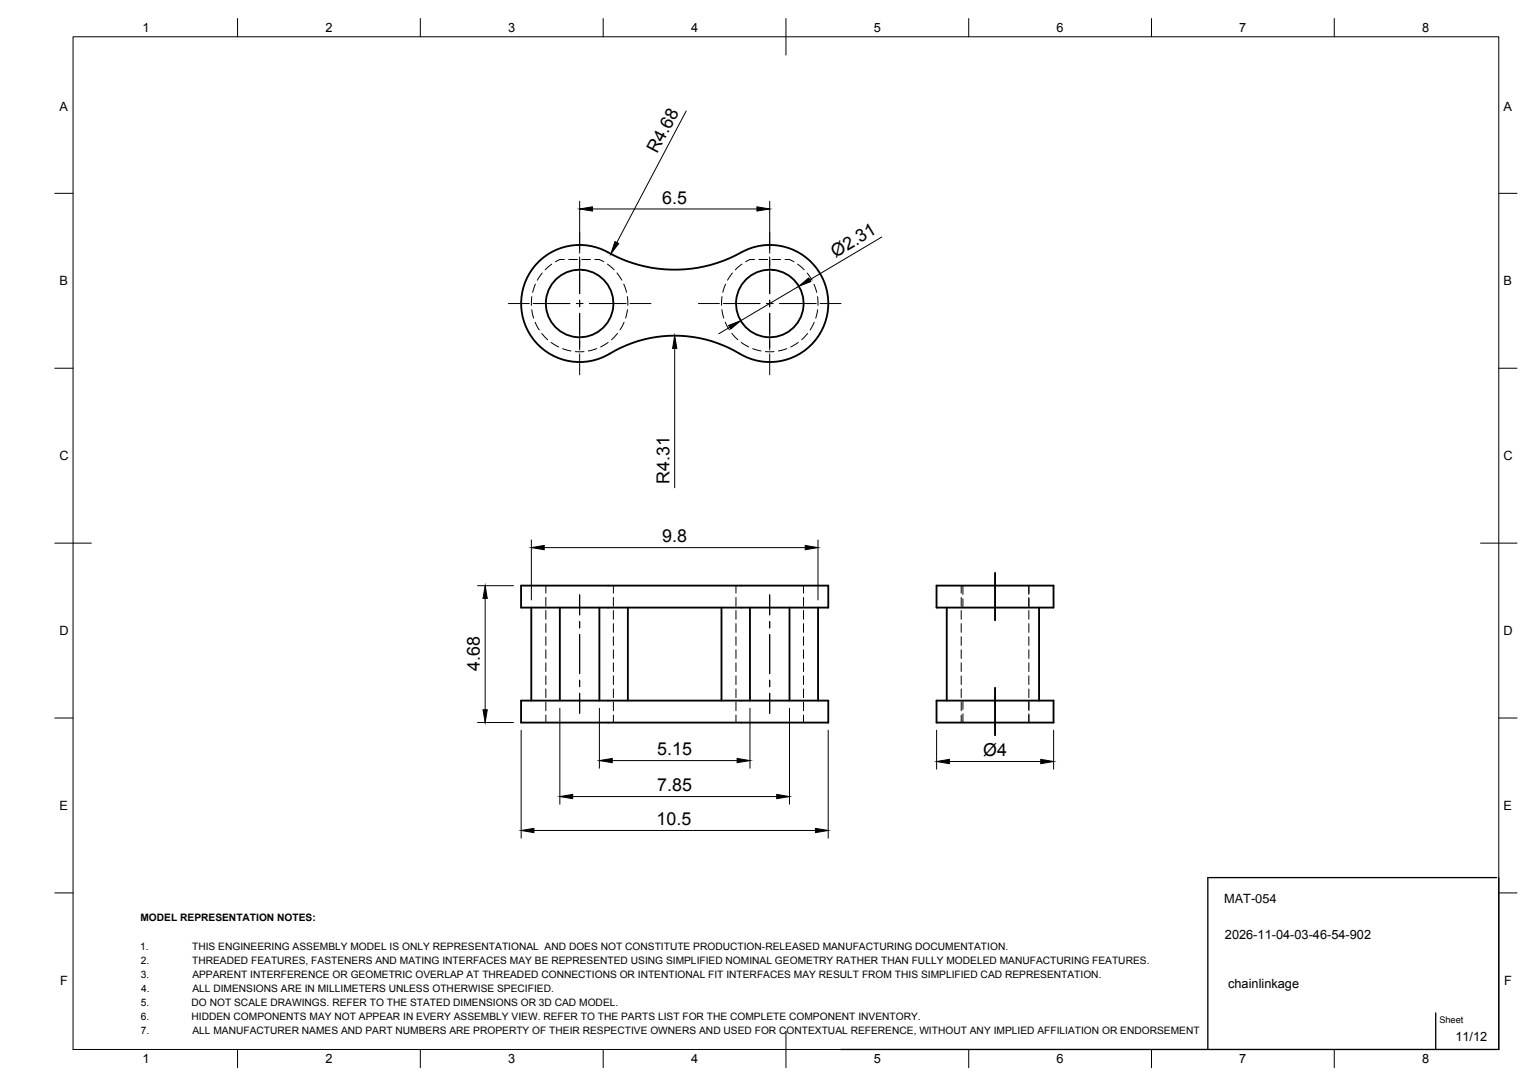
ISO-10303-21;
HEADER;
FILE_DESCRIPTION (('STEP AP214'),
    '1' );
FILE_NAME ('chainlinkage.step',
    '2026-10-21T17:50:41',
    ( '' ),
    ( '' ),
    'SwSTEP 2.0',
    'SolidWorks 2026',
    '' );
FILE_SCHEMA (( 'AUTOMOTIVE_DESIGN' ));
ENDSEC;

DATA;
#40=EDGE_CURVE ( 'NONE', #12730, #28037, #25521, .T. ) ;
#55=CIRCLE ( 'NONE', #10291, 1.154999999999999805 ) ;
#66=EDGE_CURVE ( 'NONE', #35075, #4705, #9334, .T. ) ;
#88=CARTESIAN_POINT ( 'NONE',  ( -1.030735741678193484, 1.713938105891546826, 0.000000000000000000 ) ) ;
#134=AXIS2_PLACEMENT_3D ( 'NONE', #22862, #33708, #9328 ) ;
#138=DIRECTION ( 'NONE',  ( 0.000000000000000000, 0.000000000000000000, -1.000000000000000000 ) ) ;
#168=ORIENTED_EDGE ( 'NONE', *, *, #16056, .F. ) ;
#182=LINE ( 'NONE', #27055, #31152 ) ;
#199=VERTEX_POINT ( 'NONE', #26920 ) ;
#276=DIRECTION ( 'NONE',  ( 0.000000000000000000, 0.000000000000000000, -1.000000000000000000 ) ) ;
#307=DIRECTION ( 'NONE',  ( 0.000000000000000000, 0.000000000000000000, 1.000000000000000000 ) ) ;
#314=CYLINDRICAL_SURFACE ( 'NONE', #12647, 1.649999999999999911 ) ;
#437=CARTESIAN_POINT ( 'NONE',  ( -4.850000000000000533, 0.000000000000000000, 3.180000000000000160 ) ) ;
#482=EDGE_CURVE ( 'NONE', #12038, #33286, #10560, .T. ) ;
#535=DIRECTION ( 'NONE',  ( -1.000000000000000000, 0.000000000000000000, 0.000000000000000000 ) ) ;
#566=LINE ( 'NONE', #21926, #17059 ) ;
#682=EDGE_CURVE ( 'NONE', #30822, #12038, #929, .T. ) ;
#710=LINE ( 'NONE', #3191, #33103 ) ;
#771=ORIENTED_EDGE ( 'NONE', *, *, #682, .T. ) ;
#821=CYLINDRICAL_SURFACE ( 'NONE', #2018, 1.155000000000000027 ) ;
#827=MANIFOLD_SOLID_BREP ( 'Cut-Extrude2', #21909 ) ;
#929=CIRCLE ( 'NONE', #2617, 1.999999999999999112 ) ;
#964=CARTESIAN_POINT ( 'NONE',  ( -3.250000000000000000, 5.404196845913421754, 3.180000000000000160 ) ) ;
#985=PRODUCT ( 'chainlinkage', 'chainlinkage', '', ( #30098 ) ) ;
#989=ORIENTED_EDGE ( 'NONE', *, *, #16056, .T. ) ;
#991=AXIS2_PLACEMENT_3D ( 'NONE', #11970, #9804, #22814 ) ;
#1064=EDGE_CURVE ( 'NONE', #21836, #5569, #31063, .T. ) ;
#1066=ORIENTED_EDGE ( 'NONE', *, *, #40, .F. ) ;
#1108=AXIS2_PLACEMENT_3D ( 'NONE', #964, #6635, #11836 ) ;
#1198=CARTESIAN_POINT ( 'NONE',  ( 0.000000000000000000, 0.000000000000000000, -0.7500000000000000000 ) ) ;
#1209=DIRECTION ( 'NONE',  ( -0.000000000000000000, -0.000000000000000000, 1.000000000000000000 ) ) ;
#1225=CYLINDRICAL_SURFACE ( 'NONE', #27765, 4.306175033202026547 ) ;
#1325=CYLINDRICAL_SURFACE ( 'NONE', #28033, 4.682234377621698584 ) ;
#1361=AXIS2_PLACEMENT_3D ( 'NONE', #8984, #1501, #28384 ) ;
#1377=DIRECTION ( 'NONE',  ( -1.000000000000000000, 0.000000000000000000, 0.000000000000000000 ) ) ;
#1400=FACE_OUTER_BOUND ( 'NONE', #34513, .T. ) ;
#1435=ORIENTED_EDGE ( 'NONE', *, *, #66, .T. ) ;
#1439=EDGE_CURVE ( 'NONE', #23165, #2399, #29356, .T. ) ;
#1450=DIRECTION ( 'NONE',  ( -1.000000000000000000, 0.000000000000000000, 0.000000000000000000 ) ) ;
#1454=ADVANCED_FACE ( 'NONE', ( #13767, #18767, #5385 ), #5722, .F. ) ;
#1484=DIRECTION ( 'NONE',  ( -0.000000000000000000, -0.000000000000000000, -1.000000000000000000 ) ) ;
#1494=DIRECTION ( 'NONE',  ( -1.000000000000000000, 0.000000000000000000, 0.000000000000000000 ) ) ;
#1501=DIRECTION ( 'NONE',  ( 0.000000000000000000, 0.000000000000000000, 1.000000000000000000 ) ) ;
#1503=CARTESIAN_POINT ( 'NONE',  ( 1.649999999999999911, 2.020667218593132262E-16, 3.180000000000000160 ) ) ;
#1508=AXIS2_PLACEMENT_3D ( 'NONE', #34955, #16626, #13943 ) ;
#1527=ORIENTED_EDGE ( 'NONE', *, *, #26835, .F. ) ;
#1649=FACE_OUTER_BOUND ( 'NONE', #18770, .T. ) ;
#1716=VERTEX_POINT ( 'NONE', #4860 ) ;
#1878=AXIS2_PLACEMENT_3D ( 'NONE', #8187, #21720, #29213 ) ;
#1888=CARTESIAN_POINT ( 'NONE',  ( -7.654999999999999361, 0.000000000000000000, -0.7500000000000000000 ) ) ;
#1966=DIRECTION ( 'NONE',  ( 0.000000000000000000, 0.000000000000000000, 1.000000000000000000 ) ) ;
#1967=DIRECTION ( 'NONE',  ( -0.000000000000000000, -0.000000000000000000, -1.000000000000000000 ) ) ;
#1984=FACE_OUTER_BOUND ( 'NONE', #24660, .T. ) ;
#2018=AXIS2_PLACEMENT_3D ( 'NONE', #25544, #30893, #9697 ) ;
#2045=DIRECTION ( 'NONE',  ( -0.000000000000000000, -0.000000000000000000, 1.000000000000000000 ) ) ;
#2069=CARTESIAN_POINT ( 'NONE',  ( 0.000000000000000000, 0.000000000000000000, 3.180000000000000160 ) ) ;
#2084=CARTESIAN_POINT ( 'NONE',  ( -1.155000000000000027, 0.000000000000000000, 3.931000000000000494 ) ) ;
#2200=DIRECTION ( 'NONE',  ( 0.000000000000000000, 0.000000000000000000, 1.000000000000000000 ) ) ;
#2204=AXIS2_PLACEMENT_3D ( 'NONE', #21496, #307, #5793 ) ;
#2302=CARTESIAN_POINT ( 'NONE',  ( -1.649999999999999911, 0.000000000000000000, 0.000000000000000000 ) ) ;
#2344=CARTESIAN_POINT ( 'NONE',  ( -7.176301005103106867, -1.505030548027689097, 3.180000000000000160 ) ) ;
#2394=ORIENTED_EDGE ( 'NONE', *, *, #29927, .T. ) ;
#2399=VERTEX_POINT ( 'NONE', #33596 ) ;
#2472=EDGE_CURVE ( 'NONE', #12505, #8625, #18135, .T. ) ;
#2502=CIRCLE ( 'NONE', #7660, 1.154999999999999805 ) ;
#2514=EDGE_CURVE ( 'NONE', #18417, #33401, #8920, .T. ) ;
#2580=ORIENTED_EDGE ( 'NONE', *, *, #29927, .F. ) ;
#2602=ORIENTED_EDGE ( 'NONE', *, *, #7802, .F. ) ;
#2615=FACE_BOUND ( 'NONE', #28818, .T. ) ;
#2617=AXIS2_PLACEMENT_3D ( 'NONE', #29913, #32389, #29730 ) ;
#2676=AXIS2_PLACEMENT_3D ( 'NONE', #27749, #22602, #25066 ) ;
#2729=VERTEX_POINT ( 'NONE', #4345 ) ;
#2774=ADVANCED_FACE ( 'NONE', ( #20561 ), #821, .F. ) ;
#2818=ORIENTED_EDGE ( 'NONE', *, *, #9035, .F. ) ;
#2860=DIRECTION ( 'NONE',  ( 0.000000000000000000, 0.000000000000000000, 1.000000000000000000 ) ) ;
#2899=DIRECTION ( 'NONE',  ( -0.000000000000000000, -0.000000000000000000, 1.000000000000000000 ) ) ;
#2914=AXIS2_PLACEMENT_3D ( 'NONE', #6195, #27746, #21882 ) ;
#2938=CIRCLE ( 'NONE', #11474, 4.306175033202026547 ) ;
#3041=LINE ( 'NONE', #24925, #28895 ) ;
#3082=AXIS2_PLACEMENT_3D ( 'NONE', #22310, #2899, #30499 ) ;
#3134=FACE_OUTER_BOUND ( 'NONE', #25988, .T. ) ;
#3143=AXIS2_PLACEMENT_3D ( 'NONE', #3833, #12401, #9707 ) ;
#3191=CARTESIAN_POINT ( 'NONE',  ( -7.176301005103106867, -1.505030548027689319, -0.7520000000000004459 ) ) ;
#3223=CARTESIAN_POINT ( 'NONE',  ( -1.030735741678193262, 1.713938105891546382, 3.180000000000000160 ) ) ;
#3254=ORIENTED_EDGE ( 'NONE', *, *, #5133, .T. ) ;
#3318=CARTESIAN_POINT ( 'NONE',  ( -7.654999999999999361, 0.000000000000000000, 3.930000000000000160 ) ) ;
#3324=EDGE_CURVE ( 'NONE', #3609, #8625, #6118, .T. ) ;
#3348=VERTEX_POINT ( 'NONE', #34569 ) ;
#3431=ORIENTED_EDGE ( 'NONE', *, *, #482, .F. ) ;
#3446=EDGE_CURVE ( 'NONE', #27961, #23165, #3041, .T. ) ;
#3464=CIRCLE ( 'NONE', #27913, 1.154999999999999805 ) ;
#3503=VERTEX_POINT ( 'NONE', #24569 ) ;
#3515=ADVANCED_FACE ( 'NONE', ( #13394, #24227, #21920 ), #27431, .F. ) ;
#3579=CARTESIAN_POINT ( 'NONE',  ( -3.250000000000000000, -5.838643359331793015, 0.000000000000000000 ) ) ;
#3605=ORIENTED_EDGE ( 'NONE', *, *, #21510, .T. ) ;
#3609=VERTEX_POINT ( 'NONE', #14453 ) ;
#3789=DIRECTION ( 'NONE',  ( 1.000000000000000000, 0.000000000000000000, 0.000000000000000000 ) ) ;
#3812=ORIENTED_EDGE ( 'NONE', *, *, #482, .T. ) ;
#3833=CARTESIAN_POINT ( 'NONE',  ( -6.500000000000000000, 0.000000000000000000, 0.000000000000000000 ) ) ;
#3873=AXIS2_PLACEMENT_3D ( 'NONE', #5358, #13399, #18913 ) ;
#3951=ORIENTED_EDGE ( 'NONE', *, *, #4235, .F. ) ;
#3972=DIRECTION ( 'NONE',  ( -0.000000000000000000, -0.000000000000000000, -1.000000000000000000 ) ) ;
#4059=AXIS2_PLACEMENT_3D ( 'NONE', #34539, #31851, #1450 ) ;
#4090=ORIENTED_EDGE ( 'NONE', *, *, #26835, .T. ) ;
#4100=DIRECTION ( 'NONE',  ( 1.000000000000000000, 0.000000000000000000, 0.000000000000000000 ) ) ;
#4113=SHAPE_REPRESENTATION_RELATIONSHIP ( 'NONE' , 'NONE' ,  #28231, #21564 ) ;
#4120=ORIENTED_EDGE ( 'NONE', *, *, #30868, .F. ) ;
#4146=FACE_OUTER_BOUND ( 'NONE', #31362, .T. ) ;
#4172=AXIS2_PLACEMENT_3D ( 'NONE', #31624, #1209, #20777 ) ;
#4235=EDGE_CURVE ( 'NONE', #29254, #3503, #20422, .T. ) ;
#4274=DIRECTION ( 'NONE',  ( 0.000000000000000000, 0.000000000000000000, 1.000000000000000000 ) ) ;
#4309=DIRECTION ( 'NONE',  ( 1.000000000000000000, 0.000000000000000000, 0.000000000000000000 ) ) ;
#4345=CARTESIAN_POINT ( 'NONE',  ( -5.469264258321805627, 1.713938105891546382, 0.000000000000000000 ) ) ;
#4391=ORIENTED_EDGE ( 'NONE', *, *, #15235, .F. ) ;
#4398=EDGE_CURVE ( 'NONE', #4705, #20910, #34075, .T. ) ;
#4416=CIRCLE ( 'NONE', #28250, 1.649999999999999467 ) ;
#4437=DIRECTION ( 'NONE',  ( -0.000000000000000000, -0.000000000000000000, -1.000000000000000000 ) ) ;
#4501=CARTESIAN_POINT ( 'NONE',  ( 0.000000000000000000, 0.000000000000000000, 3.930000000000000160 ) ) ;
#4599=CARTESIAN_POINT ( 'NONE',  ( -5.344999999999999751, 1.414467053015192657E-16, 3.931000000000000494 ) ) ;
#4656=AXIS2_PLACEMENT_3D ( 'NONE', #22342, #8808, #10646 ) ;
#4664=ORIENTED_EDGE ( 'NONE', *, *, #22172, .F. ) ;
#4673=ORIENTED_EDGE ( 'NONE', *, *, #5133, .F. ) ;
#4705=VERTEX_POINT ( 'NONE', #3223 ) ;
#4730=CIRCLE ( 'NONE', #1361, 1.649999999999999911 ) ;
#4740=EDGE_CURVE ( 'NONE', #29809, #23630, #11916, .T. ) ;
#4749=CYLINDRICAL_SURFACE ( 'NONE', #23978, 4.682234377621698584 ) ;
#4756=DIRECTION ( 'NONE',  ( 1.000000000000000000, 0.000000000000000000, 0.000000000000000000 ) ) ;
#4767=EDGE_CURVE ( 'NONE', #33660, #29323, #566, .T. ) ;
#4826=ORIENTED_EDGE ( 'NONE', *, *, #24296, .T. ) ;
#4860=CARTESIAN_POINT ( 'NONE',  ( -0.9727285265192158192, -1.747512292859697114, 3.180000000000000160 ) ) ;
#4951=ORIENTED_EDGE ( 'NONE', *, *, #22673, .F. ) ;
#5048=ORIENTED_EDGE ( 'NONE', *, *, #9299, .F. ) ;
#5073=EDGE_LOOP ( 'NONE', ( #6133, #11536, #3605, #34483 ) ) ;
#5133=EDGE_CURVE ( 'NONE', #33286, #25337, #16417, .T. ) ;
#5167=DIRECTION ( 'NONE',  ( 0.000000000000000000, -1.000000000000000000, -0.000000000000000000 ) ) ;
#5311=DIRECTION ( 'NONE',  ( -1.000000000000000000, 0.000000000000000000, 0.000000000000000000 ) ) ;
#5331=DIRECTION ( 'NONE',  ( -0.000000000000000000, -0.000000000000000000, 1.000000000000000000 ) ) ;
#5340=ORIENTED_EDGE ( 'NONE', *, *, #6899, .T. ) ;
#5358=CARTESIAN_POINT ( 'NONE',  ( -6.500000000000000000, 0.000000000000000000, 0.000000000000000000 ) ) ;
#5385=FACE_OUTER_BOUND ( 'NONE', #19054, .T. ) ;
#5440=ADVANCED_FACE ( 'NONE', ( #5955 ), #24299, .T. ) ;
#5460=FACE_OUTER_BOUND ( 'NONE', #18521, .T. ) ;
#5494=ORIENTED_EDGE ( 'NONE', *, *, #66, .F. ) ;
#5519=DIRECTION ( 'NONE',  ( -1.000000000000000000, 0.000000000000000000, 0.000000000000000000 ) ) ;
#5569=VERTEX_POINT ( 'NONE', #28408 ) ;
#5722=PLANE ( 'NONE',  #1508 ) ;
#5770=ADVANCED_FACE ( 'NONE', ( #7543 ), #24568, .T. ) ;
#5793=DIRECTION ( 'NONE',  ( 1.000000000000000000, 0.000000000000000000, -0.000000000000000000 ) ) ;
#5798=VECTOR ( 'NONE', #23744, 1000.000000000000000 ) ;
#5931=DIRECTION ( 'NONE',  ( -0.000000000000000000, -0.000000000000000000, -1.000000000000000000 ) ) ;
#5955=FACE_OUTER_BOUND ( 'NONE', #5073, .T. ) ;
#6045=AXIS2_PLACEMENT_3D ( 'NONE', #20829, #26336, #18181 ) ;
#6058=CARTESIAN_POINT ( 'NONE',  ( -5.527271473480783293, -1.747512292859696226, 3.930000000000000160 ) ) ;
#6059=DIRECTION ( 'NONE',  ( 1.000000000000000000, 0.000000000000000000, 0.000000000000000000 ) ) ;
#6118=CIRCLE ( 'NONE', #19790, 1.155000000000000027 ) ;
#6133=ORIENTED_EDGE ( 'NONE', *, *, #12186, .T. ) ;
#6145=CYLINDRICAL_SURFACE ( 'NONE', #28870, 1.154999999999999805 ) ;
#6165=EDGE_CURVE ( 'NONE', #28037, #17552, #2502, .T. ) ;
#6195=CARTESIAN_POINT ( 'NONE',  ( -6.500000000000000000, 0.000000000000000000, 3.180000000000000160 ) ) ;
#6236=LINE ( 'NONE', #31639, #19124 ) ;
#6282=DIRECTION ( 'NONE',  ( 0.000000000000000000, 0.000000000000000000, -1.000000000000000000 ) ) ;
#6300=DIRECTION ( 'NONE',  ( -1.000000000000000000, 0.000000000000000000, 0.000000000000000000 ) ) ;
#6416=( GEOMETRIC_REPRESENTATION_CONTEXT ( 3 ) GLOBAL_UNCERTAINTY_ASSIGNED_CONTEXT ( ( #12114 ) ) GLOBAL_UNIT_ASSIGNED_CONTEXT ( ( #20850, #12680, #7306 ) ) REPRESENTATION_CONTEXT ( 'NONE', 'WORKASPACE' ) );
#6454=CARTESIAN_POINT ( 'NONE',  ( -8.499999999999998224, 0.000000000000000000, 3.930000000000000160 ) ) ;
#6553=DIRECTION ( 'NONE',  ( 0.000000000000000000, -0.000000000000000000, 1.000000000000000000 ) ) ;
#6635=DIRECTION ( 'NONE',  ( -0.000000000000000000, -0.000000000000000000, -1.000000000000000000 ) ) ;
#6684=CYLINDRICAL_SURFACE ( 'NONE', #20583, 1.155000000000000027 ) ;
#6696=ORIENTED_EDGE ( 'NONE', *, *, #13553, .T. ) ;
#6733=ORIENTED_EDGE ( 'NONE', *, *, #29169, .T. ) ;
#6740=CARTESIAN_POINT ( 'NONE',  ( -5.823698994896893133, -1.505030548027689319, -0.7520000000000004459 ) ) ;
#6791=ORIENTED_EDGE ( 'NONE', *, *, #21853, .F. ) ;
#6899=EDGE_CURVE ( 'NONE', #22009, #199, #18522, .T. ) ;
#6912=CARTESIAN_POINT ( 'NONE',  ( -1.030735741678193484, 1.713938105891546826, -0.7500000000000000000 ) ) ;
#6929=CIRCLE ( 'NONE', #30157, 1.155000000000000027 ) ;
#6967=EDGE_LOOP ( 'NONE', ( #10488, #18063 ) ) ;
#7038=ORIENTED_EDGE ( 'NONE', *, *, #8514, .F. ) ;
#7071=CARTESIAN_POINT ( 'NONE',  ( -8.149999999999998579, 2.020667218593132508E-16, -0.7520000000000004459 ) ) ;
#7141=ORIENTED_EDGE ( 'NONE', *, *, #22646, .T. ) ;
#7147=ORIENTED_EDGE ( 'NONE', *, *, #4740, .T. ) ;
#7199=VERTEX_POINT ( 'NONE', #27130 ) ;
#7207=EDGE_CURVE ( 'NONE', #29809, #21836, #24442, .T. ) ;
#7306=( NAMED_UNIT ( * ) SI_UNIT ( $, .STERADIAN. ) SOLID_ANGLE_UNIT ( ) );
#7310=PLANE ( 'NONE',  #30127 ) ;
#7313=VERTEX_POINT ( 'NONE', #17881 ) ;
#7404=CARTESIAN_POINT ( 'NONE',  ( 0.000000000000000000, 0.000000000000000000, -0.7500000000000000000 ) ) ;
#7492=ORIENTED_EDGE ( 'NONE', *, *, #32135, .F. ) ;
#7543=FACE_OUTER_BOUND ( 'NONE', #29636, .T. ) ;
#7594=CARTESIAN_POINT ( 'NONE',  ( -1.155000000000000027, 0.000000000000000000, 3.930000000000000160 ) ) ;
#7660=AXIS2_PLACEMENT_3D ( 'NONE', #29186, #26509, #5311 ) ;
#7663=VECTOR ( 'NONE', #34331, 1000.000000000000000 ) ;
#7708=AXIS2_PLACEMENT_3D ( 'NONE', #11779, #33468, #22629 ) ;
#7764=ORIENTED_EDGE ( 'NONE', *, *, #16575, .T. ) ;
#7780=CARTESIAN_POINT ( 'NONE',  ( -5.527271473480783293, -1.747512292859696226, 3.180000000000000160 ) ) ;
#7792=VECTOR ( 'NONE', #28961, 1000.000000000000000 ) ;
#7797=AXIS2_PLACEMENT_3D ( 'NONE', #16325, #27324, #27681 ) ;
#7802=EDGE_CURVE ( 'NONE', #7313, #3609, #6236, .T. ) ;
#7907=ORIENTED_EDGE ( 'NONE', *, *, #18077, .T. ) ;
#7936=ORIENTED_EDGE ( 'NONE', *, *, #11972, .T. ) ;
#8100=AXIS2_PLACEMENT_3D ( 'NONE', #4501, #10215, #17430 ) ;
#8187=CARTESIAN_POINT ( 'NONE',  ( 0.000000000000000000, 0.000000000000000000, -0.7500000000000000000 ) ) ;
#8321=CARTESIAN_POINT ( 'NONE',  ( 0.6763010051031078662, -1.505030548027689319, 3.180000000000000160 ) ) ;
#8322=DIRECTION ( 'NONE',  ( 0.000000000000000000, -1.000000000000000000, -0.000000000000000000 ) ) ;
#8389=DIRECTION ( 'NONE',  ( -1.000000000000000000, 0.000000000000000000, -0.000000000000000000 ) ) ;
#8415=CARTESIAN_POINT ( 'NONE',  ( -0.9727285265192158192, -1.747512292859697114, 3.930000000000000160 ) ) ;
#8485=EDGE_CURVE ( 'NONE', #29323, #2729, #14525, .T. ) ;
#8514=EDGE_CURVE ( 'NONE', #12038, #10814, #22512, .T. ) ;
#8557=DIRECTION ( 'NONE',  ( 0.000000000000000000, 0.000000000000000000, -1.000000000000000000 ) ) ;
#8625=VERTEX_POINT ( 'NONE', #25877 ) ;
#8711=CARTESIAN_POINT ( 'NONE',  ( -5.469264258321805627, 1.713938105891546382, -0.7500000000000000000 ) ) ;
#8748=DIRECTION ( 'NONE',  ( 1.000000000000000000, 0.000000000000000000, 0.000000000000000000 ) ) ;
#8774=CIRCLE ( 'NONE', #3082, 4.306175033202026547 ) ;
#8807=ORIENTED_EDGE ( 'NONE', *, *, #8485, .T. ) ;
#8808=DIRECTION ( 'NONE',  ( -0.000000000000000000, -0.000000000000000000, -1.000000000000000000 ) ) ;
#8832=CARTESIAN_POINT ( 'NONE',  ( 0.000000000000000000, 0.000000000000000000, 3.931000000000000494 ) ) ;
#8918=EDGE_LOOP ( 'NONE', ( #32736, #5494, #2818, #23655 ) ) ;
#8920=CIRCLE ( 'NONE', #28813, 1.999999999999999556 ) ;
#8984=CARTESIAN_POINT ( 'NONE',  ( 0.000000000000000000, 0.000000000000000000, 0.000000000000000000 ) ) ;
#8995=EDGE_CURVE ( 'NONE', #17552, #28037, #26007, .T. ) ;
#9035=EDGE_CURVE ( 'NONE', #25337, #35075, #21466, .T. ) ;
#9049=ORIENTED_EDGE ( 'NONE', *, *, #13553, .F. ) ;
#9104=CARTESIAN_POINT ( 'NONE',  ( -6.500000000000000000, 0.000000000000000000, 3.180000000000000160 ) ) ;
#9107=DIRECTION ( 'NONE',  ( -1.000000000000000000, 0.000000000000000000, 0.000000000000000000 ) ) ;
#9121=EDGE_CURVE ( 'NONE', #18796, #29323, #12382, .T. ) ;
#9130=ORIENTED_EDGE ( 'NONE', *, *, #2514, .F. ) ;
#9133=VECTOR ( 'NONE', #25196, 1000.000000000000000 ) ;
#9150=DIRECTION ( 'NONE',  ( -0.000000000000000000, -0.000000000000000000, -1.000000000000000000 ) ) ;
#9201=EDGE_LOOP ( 'NONE', ( #10758, #13153, #14179, #4391 ) ) ;
#9299=EDGE_CURVE ( 'NONE', #33401, #21805, #182, .T. ) ;
#9328=DIRECTION ( 'NONE',  ( 1.000000000000000000, 0.000000000000000000, 0.000000000000000000 ) ) ;
#9332=DIRECTION ( 'NONE',  ( -1.000000000000000000, 0.000000000000000000, 0.000000000000000000 ) ) ;
#9334=LINE ( 'NONE', #24985, #34981 ) ;
#9365=ORIENTED_EDGE ( 'NONE', *, *, #1439, .F. ) ;
#9411=VERTEX_POINT ( 'NONE', #8711 ) ;
#9425=AXIS2_PLACEMENT_3D ( 'NONE', #12325, #31182, #4100 ) ;
#9447=EDGE_CURVE ( 'NONE', #7199, #33055, #30961, .T. ) ;
#9515=CARTESIAN_POINT ( 'NONE',  ( -7.654999999999999361, 0.000000000000000000, 3.931000000000000494 ) ) ;
#9548=DIRECTION ( 'NONE',  ( -0.000000000000000000, -0.000000000000000000, 1.000000000000000000 ) ) ;
#9573=DIRECTION ( 'NONE',  ( 0.000000000000000000, 0.000000000000000000, 1.000000000000000000 ) ) ;
#9640=ADVANCED_FACE ( 'NONE', ( #3134 ), #6145, .F. ) ;
#9694=AXIS2_PLACEMENT_3D ( 'NONE', #22728, #9548, #22897 ) ;
#9697=DIRECTION ( 'NONE',  ( -1.000000000000000000, 0.000000000000000000, 0.000000000000000000 ) ) ;
#9707=DIRECTION ( 'NONE',  ( -1.000000000000000000, 0.000000000000000000, 0.000000000000000000 ) ) ;
#9741=FACE_OUTER_BOUND ( 'NONE', #14669, .T. ) ;
#9799=CARTESIAN_POINT ( 'NONE',  ( -4.850000000000000533, 0.000000000000000000, 0.000000000000000000 ) ) ;
#9804=DIRECTION ( 'NONE',  ( 0.000000000000000000, 0.000000000000000000, -1.000000000000000000 ) ) ;
#9830=DIRECTION ( 'NONE',  ( -0.000000000000000000, -0.000000000000000000, -1.000000000000000000 ) ) ;
#9856=DIRECTION ( 'NONE',  ( 1.000000000000000000, 0.000000000000000000, 0.000000000000000000 ) ) ;
#9949=LINE ( 'NONE', #6912, #7663 ) ;
#10090=ORIENTED_EDGE ( 'NONE', *, *, #9447, .T. ) ;
#10115=ORIENTED_EDGE ( 'NONE', *, *, #18665, .T. ) ;
#10215=DIRECTION ( 'NONE',  ( -0.000000000000000000, -0.000000000000000000, -1.000000000000000000 ) ) ;
#10291=AXIS2_PLACEMENT_3D ( 'NONE', #12003, #1484, #4309 ) ;
#10309=APPLICATION_CONTEXT ( 'automotive_design' ) ;
#10382=CARTESIAN_POINT ( 'NONE',  ( 0.000000000000000000, 0.000000000000000000, 3.180000000000000160 ) ) ;
#10488=ORIENTED_EDGE ( 'NONE', *, *, #23625, .T. ) ;
#10520=CARTESIAN_POINT ( 'NONE',  ( 1.999999999999999556, 0.000000000000000000, -0.7500000000000000000 ) ) ;
#10560=CIRCLE ( 'NONE', #9425, 1.999999999999999112 ) ;
#10630=DIRECTION ( 'NONE',  ( -1.000000000000000000, 0.000000000000000000, 0.000000000000000000 ) ) ;
#10643=AXIS2_PLACEMENT_3D ( 'NONE', #30956, #33446, #535 ) ;
#10646=DIRECTION ( 'NONE',  ( -1.000000000000000000, 0.000000000000000000, 0.000000000000000000 ) ) ;
#10758=ORIENTED_EDGE ( 'NONE', *, *, #4740, .F. ) ;
#10814=VERTEX_POINT ( 'NONE', #30101 ) ;
#10915=DIRECTION ( 'NONE',  ( 0.000000000000000000, 0.000000000000000000, 1.000000000000000000 ) ) ;
#10926=ORIENTED_EDGE ( 'NONE', *, *, #20454, .T. ) ;
#10931=CIRCLE ( 'NONE', #134, 1.649999999999999911 ) ;
#11145=EDGE_LOOP ( 'NONE', ( #15185, #4090, #7147, #34207 ) ) ;
#11156=ORIENTED_EDGE ( 'NONE', *, *, #35061, .F. ) ;
#11226=( NAMED_UNIT ( * ) PLANE_ANGLE_UNIT ( ) SI_UNIT ( $, .RADIAN. ) );
#11352=AXIS2_PLACEMENT_3D ( 'NONE', #13439, #20914, #15771 ) ;
#11474=AXIS2_PLACEMENT_3D ( 'NONE', #33239, #25216, #14393 ) ;
#11478=DIRECTION ( 'NONE',  ( -1.000000000000000000, 0.000000000000000000, 0.000000000000000000 ) ) ;
#11489=CYLINDRICAL_SURFACE ( 'NONE', #4656, 1.999999999999999112 ) ;
#11515=CYLINDRICAL_SURFACE ( 'NONE', #9694, 1.999999999999999112 ) ;
#11523=CIRCLE ( 'NONE', #8100, 1.155000000000000027 ) ;
#11536=ORIENTED_EDGE ( 'NONE', *, *, #35061, .T. ) ;
#11591=ORIENTED_EDGE ( 'NONE', *, *, #1064, .F. ) ;
#11779=CARTESIAN_POINT ( 'NONE',  ( -6.500000000000000000, 0.000000000000000000, 0.000000000000000000 ) ) ;
#11810=CARTESIAN_POINT ( 'NONE',  ( 0.000000000000000000, 0.000000000000000000, 3.930000000000000160 ) ) ;
#11836=DIRECTION ( 'NONE',  ( 1.000000000000000000, 0.000000000000000000, 0.000000000000000000 ) ) ;
#11843=ORIENTED_EDGE ( 'NONE', *, *, #21898, .T. ) ;
#11916=CIRCLE ( 'NONE', #33493, 1.649999999999999911 ) ;
#11970=CARTESIAN_POINT ( 'NONE',  ( -6.500000000000000000, 0.000000000000000000, -0.7500000000000000000 ) ) ;
#11971=CARTESIAN_POINT ( 'NONE',  ( 0.000000000000000000, 0.000000000000000000, -0.7500000000000000000 ) ) ;
#11972=EDGE_CURVE ( 'NONE', #33055, #29254, #30854, .T. ) ;
#12003=CARTESIAN_POINT ( 'NONE',  ( -6.500000000000000000, 0.000000000000000000, 3.930000000000000160 ) ) ;
#12016=DIRECTION ( 'NONE',  ( -0.000000000000000000, -0.000000000000000000, -1.000000000000000000 ) ) ;
#12023=DIRECTION ( 'NONE',  ( -0.000000000000000000, -0.000000000000000000, -1.000000000000000000 ) ) ;
#12038=VERTEX_POINT ( 'NONE', #6454 ) ;
#12076=DIRECTION ( 'NONE',  ( -0.000000000000000000, -0.000000000000000000, 1.000000000000000000 ) ) ;
#12114=UNCERTAINTY_MEASURE_WITH_UNIT (LENGTH_MEASURE( 1.000000000000000082E-05 ), #20850, 'distance_accuracy_value', 'NONE');
#12154=DIRECTION ( 'NONE',  ( -0.000000000000000000, -0.000000000000000000, -1.000000000000000000 ) ) ;
#12168=AXIS2_PLACEMENT_3D ( 'NONE', #12667, #1967, #21016 ) ;
#12171=EDGE_LOOP ( 'NONE', ( #5048, #9130, #19712, #14712 ) ) ;
#12186=EDGE_CURVE ( 'NONE', #7199, #29588, #15848, .T. ) ;
#12203=DIRECTION ( 'NONE',  ( -0.000000000000000000, -0.000000000000000000, -1.000000000000000000 ) ) ;
#12232=DIRECTION ( 'NONE',  ( -1.000000000000000000, 0.000000000000000000, 0.000000000000000000 ) ) ;
#12256=CARTESIAN_POINT ( 'NONE',  ( -6.500000000000000000, 0.000000000000000000, 3.180000000000000160 ) ) ;
#12325=CARTESIAN_POINT ( 'NONE',  ( -6.500000000000000000, 0.000000000000000000, 3.930000000000000160 ) ) ;
#12382=CIRCLE ( 'NONE', #24264, 4.682234377621698584 ) ;
#12401=DIRECTION ( 'NONE',  ( -0.000000000000000000, -0.000000000000000000, 1.000000000000000000 ) ) ;
#12412=VECTOR ( 'NONE', #25783, 1000.000000000000000 ) ;
#12433=ADVANCED_FACE ( 'NONE', ( #1400 ), #1225, .F. ) ;
#12505=VERTEX_POINT ( 'NONE', #7594 ) ;
#12588=ADVANCED_FACE ( 'NONE', ( #2615, #13483, #24484 ), #13319, .T. ) ;
#12619=VECTOR ( 'NONE', #30124, 1000.000000000000000 ) ;
#12647=AXIS2_PLACEMENT_3D ( 'NONE', #30382, #19192, #14202 ) ;
#12658=ORIENTED_EDGE ( 'NONE', *, *, #12186, .F. ) ;
#12667=CARTESIAN_POINT ( 'NONE',  ( -3.250000000000000000, 5.404196845913421754, 3.930000000000000160 ) ) ;
#12680=( NAMED_UNIT ( * ) PLANE_ANGLE_UNIT ( ) SI_UNIT ( $, .RADIAN. ) );
#12730=VERTEX_POINT ( 'NONE', #3318 ) ;
#12752=CIRCLE ( 'NONE', #34329, 1.999999999999999556 ) ;
#12872=DIRECTION ( 'NONE',  ( -1.000000000000000000, 0.000000000000000000, 0.000000000000000000 ) ) ;
#12883=DIRECTION ( 'NONE',  ( -1.000000000000000000, 0.000000000000000000, 0.000000000000000000 ) ) ;
#13073=DIRECTION ( 'NONE',  ( 1.000000000000000000, 0.000000000000000000, 0.000000000000000000 ) ) ;
#13153=ORIENTED_EDGE ( 'NONE', *, *, #7207, .T. ) ;
#13181=AXIS2_PLACEMENT_3D ( 'NONE', #18019, #1966, #21015 ) ;
#13182=EDGE_CURVE ( 'NONE', #22127, #21805, #26672, .T. ) ;
#13261=DIRECTION ( 'NONE',  ( 1.000000000000000000, 0.000000000000000000, 0.000000000000000000 ) ) ;
#13319=PLANE ( 'NONE',  #2204 ) ;
#13394=FACE_BOUND ( 'NONE', #27036, .T. ) ;
#13399=DIRECTION ( 'NONE',  ( -0.000000000000000000, -0.000000000000000000, 1.000000000000000000 ) ) ;
#13439=CARTESIAN_POINT ( 'NONE',  ( -6.500000000000000000, 0.000000000000000000, 3.180000000000000160 ) ) ;
#13465=ORIENTED_EDGE ( 'NONE', *, *, #4767, .F. ) ;
#13483=FACE_BOUND ( 'NONE', #6967, .T. ) ;
#13496=CARTESIAN_POINT ( 'NONE',  ( 10.00000000000000000, -1.505030548027689319, 3.180000000000000160 ) ) ;
#13553=EDGE_CURVE ( 'NONE', #20910, #10814, #14215, .T. ) ;
#13595=ORIENTED_EDGE ( 'NONE', *, *, #13182, .F. ) ;
#13767=FACE_BOUND ( 'NONE', #28107, .T. ) ;
#13774=ORIENTED_EDGE ( 'NONE', *, *, #21049, .T. ) ;
#13828=ADVANCED_FACE ( 'NONE', ( #1984 ), #7310, .T. ) ;
#13885=CARTESIAN_POINT ( 'NONE',  ( 1.999999999999999556, 0.000000000000000000, 0.000000000000000000 ) ) ;
#13901=AXIS2_PLACEMENT_3D ( 'NONE', #18097, #2045, #18255 ) ;
#13943=DIRECTION ( 'NONE',  ( 1.000000000000000000, 0.000000000000000000, -0.000000000000000000 ) ) ;
#13975=ORIENTED_EDGE ( 'NONE', *, *, #19990, .T. ) ;
#14006=CARTESIAN_POINT ( 'NONE',  ( -6.500000000000000000, 0.000000000000000000, 3.931000000000000494 ) ) ;
#14015=EDGE_CURVE ( 'NONE', #33660, #9411, #16505, .T. ) ;
#14016=AXIS2_PLACEMENT_3D ( 'NONE', #34244, #31398, #9856 ) ;
#14090=CARTESIAN_POINT ( 'NONE',  ( -1.030735741678193484, 1.713938105891546826, -0.7500000000000000000 ) ) ;
#14096=ORIENTED_EDGE ( 'NONE', *, *, #21898, .F. ) ;
#14116=ORIENTED_EDGE ( 'NONE', *, *, #22646, .F. ) ;
#14179=ORIENTED_EDGE ( 'NONE', *, *, #1064, .T. ) ;
#14202=DIRECTION ( 'NONE',  ( -1.000000000000000000, 0.000000000000000000, 0.000000000000000000 ) ) ;
#14215=CIRCLE ( 'NONE', #15352, 1.999999999999999112 ) ;
#14275=ORIENTED_EDGE ( 'NONE', *, *, #23740, .F. ) ;
#14345=CYLINDRICAL_SURFACE ( 'NONE', #25223, 1.999999999999999556 ) ;
#14364=DIRECTION ( 'NONE',  ( -1.000000000000000000, 0.000000000000000000, 0.000000000000000000 ) ) ;
#14372=CARTESIAN_POINT ( 'NONE',  ( 10.00000000000000000, -1.505030548027689319, 0.000000000000000000 ) ) ;
#14393=DIRECTION ( 'NONE',  ( -1.000000000000000000, 0.000000000000000000, 0.000000000000000000 ) ) ;
#14444=ORIENTED_EDGE ( 'NONE', *, *, #26049, .T. ) ;
#14445=ORIENTED_EDGE ( 'NONE', *, *, #6165, .T. ) ;
#14453=CARTESIAN_POINT ( 'NONE',  ( 1.155000000000000027, 1.414467053015192904E-16, -0.7500000000000000000 ) ) ;
#14464=DIRECTION ( 'NONE',  ( -0.000000000000000000, -0.000000000000000000, -1.000000000000000000 ) ) ;
#14466=DIRECTION ( 'NONE',  ( 0.000000000000000000, -0.000000000000000000, 1.000000000000000000 ) ) ;
#14525=CIRCLE ( 'NONE', #23676, 1.999999999999999112 ) ;
#14573=ADVANCED_FACE ( 'NONE', ( #18820 ), #24308, .T. ) ;
#14602=ORIENTED_EDGE ( 'NONE', *, *, #3446, .T. ) ;
#14669=EDGE_LOOP ( 'NONE', ( #7907, #28039, #16853, #31698 ) ) ;
#14712=ORIENTED_EDGE ( 'NONE', *, *, #13182, .T. ) ;
#14847=ORIENTED_EDGE ( 'NONE', *, *, #9121, .T. ) ;
#14863=CARTESIAN_POINT ( 'NONE',  ( 10.00000000000000000, -1.505030548027689319, 0.000000000000000000 ) ) ;
#14867=VECTOR ( 'NONE', #34195, 1000.000000000000000 ) ;
#14899=LINE ( 'NONE', #14372, #9133 ) ;
#14916=DIRECTION ( 'NONE',  ( -0.000000000000000000, -0.000000000000000000, -1.000000000000000000 ) ) ;
#14943=CARTESIAN_POINT ( 'NONE',  ( -3.250000000000000000, 5.404196845913421754, 3.930000000000000160 ) ) ;
#15044=DIRECTION ( 'NONE',  ( -1.000000000000000000, 0.000000000000000000, 0.000000000000000000 ) ) ;
#15053=EDGE_CURVE ( 'NONE', #21780, #12730, #3464, .T. ) ;
#15185=ORIENTED_EDGE ( 'NONE', *, *, #1439, .T. ) ;
#15187=LINE ( 'NONE', #31877, #16017 ) ;
#15192=CIRCLE ( 'NONE', #10643, 1.999999999999999556 ) ;
#15235=EDGE_CURVE ( 'NONE', #23630, #5569, #15187, .T. ) ;
#15251=CARTESIAN_POINT ( 'NONE',  ( -0.9727285265192158192, -1.747512292859697114, 3.930000000000000160 ) ) ;
#15352=AXIS2_PLACEMENT_3D ( 'NONE', #12256, #9573, #34116 ) ;
#15367=CARTESIAN_POINT ( 'NONE',  ( -6.500000000000000000, 0.000000000000000000, -0.7520000000000004459 ) ) ;
#15428=VECTOR ( 'NONE', #12883, 1000.000000000000000 ) ;
#15433=ORIENTED_EDGE ( 'NONE', *, *, #9121, .F. ) ;
#15434=FACE_OUTER_BOUND ( 'NONE', #9201, .T. ) ;
#15587=PRODUCT_DEFINITION_FORMATION_WITH_SPECIFIED_SOURCE ( 'ANY', '', #985, .NOT_KNOWN. ) ;
#15726=AXIS2_PLACEMENT_3D ( 'NONE', #26795, #34284, #23605 ) ;
#15771=DIRECTION ( 'NONE',  ( 1.000000000000000000, 0.000000000000000000, 0.000000000000000000 ) ) ;
#15831=ORIENTED_EDGE ( 'NONE', *, *, #6165, .F. ) ;
#15848=CIRCLE ( 'NONE', #3873, 1.649999999999999467 ) ;
#15883=CARTESIAN_POINT ( 'NONE',  ( -5.469264258321805627, 1.713938105891546382, -0.7500000000000000000 ) ) ;
#15933=ADVANCED_FACE ( 'NONE', ( #19709 ), #6684, .F. ) ;
#15935=ADVANCED_FACE ( 'NONE', ( #30557 ), #11515, .T. ) ;
#16009=AXIS2_PLACEMENT_3D ( 'NONE', #11971, #25647, #9107 ) ;
#16017=VECTOR ( 'NONE', #9830, 1000.000000000000000 ) ;
#16056=EDGE_CURVE ( 'NONE', #27961, #5569, #14899, .T. ) ;
#16280=VERTEX_POINT ( 'NONE', #437 ) ;
#16307=CARTESIAN_POINT ( 'NONE',  ( -5.469264258321805627, 1.713938105891546382, 3.930000000000000160 ) ) ;
#16308=ORIENTED_EDGE ( 'NONE', *, *, #9299, .T. ) ;
#16316=EDGE_LOOP ( 'NONE', ( #7038, #33126, #17094, #6696 ) ) ;
#16325=CARTESIAN_POINT ( 'NONE',  ( -6.500000000000000000, 0.000000000000000000, -0.7520000000000004459 ) ) ;
#16417=CIRCLE ( 'NONE', #22661, 4.682234377621698584 ) ;
#16505=CIRCLE ( 'NONE', #23321, 1.999999999999999112 ) ;
#16536=CIRCLE ( 'NONE', #18241, 4.682234377621698584 ) ;
#16575=EDGE_CURVE ( 'NONE', #23165, #23630, #21045, .T. ) ;
#16590=SHAPE_DEFINITION_REPRESENTATION ( #29947, #28231 ) ;
#16626=DIRECTION ( 'NONE',  ( 0.000000000000000000, 0.000000000000000000, 1.000000000000000000 ) ) ;
#16640=ORIENTED_EDGE ( 'NONE', *, *, #8514, .T. ) ;
#16680=DIRECTION ( 'NONE',  ( -0.000000000000000000, -0.000000000000000000, -1.000000000000000000 ) ) ;
#16786=LINE ( 'NONE', #29944, #19215 ) ;
#16830=CARTESIAN_POINT ( 'NONE',  ( 10.00000000000000000, -1.505030548027689319, 3.180000000000000160 ) ) ;
#16853=ORIENTED_EDGE ( 'NONE', *, *, #24296, .F. ) ;
#17045=DIRECTION ( 'NONE',  ( -1.000000000000000000, 0.000000000000000000, 0.000000000000000000 ) ) ;
#17059=VECTOR ( 'NONE', #27259, 1000.000000000000000 ) ;
#17078=ORIENTED_EDGE ( 'NONE', *, *, #22172, .T. ) ;
#17094=ORIENTED_EDGE ( 'NONE', *, *, #25456, .T. ) ;
#17238=ADVANCED_FACE ( 'NONE', ( #9741 ), #20434, .F. ) ;
#17354=DIRECTION ( 'NONE',  ( -0.000000000000000000, -0.000000000000000000, 1.000000000000000000 ) ) ;
#17430=DIRECTION ( 'NONE',  ( 1.000000000000000000, 0.000000000000000000, 0.000000000000000000 ) ) ;
#17446=( GEOMETRIC_REPRESENTATION_CONTEXT ( 3 ) GLOBAL_UNCERTAINTY_ASSIGNED_CONTEXT ( ( #18439 ) ) GLOBAL_UNIT_ASSIGNED_CONTEXT ( ( #22430, #11226, #22076 ) ) REPRESENTATION_CONTEXT ( 'NONE', 'WORKASPACE' ) );
#17459=VECTOR ( 'NONE', #4437, 1000.000000000000000 ) ;
#17552=VERTEX_POINT ( 'NONE', #33201 ) ;
#17640=ORIENTED_EDGE ( 'NONE', *, *, #19656, .T. ) ;
#17670=CARTESIAN_POINT ( 'NONE',  ( -5.527271473480783293, -1.747512292859696226, 3.930000000000000160 ) ) ;
#17679=AXIS2_PLACEMENT_3D ( 'NONE', #32495, #16680, #10630 ) ;
#17726=ORIENTED_EDGE ( 'NONE', *, *, #7207, .F. ) ;
#17881=CARTESIAN_POINT ( 'NONE',  ( 1.155000000000000027, 1.414467053015192904E-16, 3.930000000000000160 ) ) ;
#17940=CARTESIAN_POINT ( 'NONE',  ( -5.527271473480783293, -1.747512292859696226, -0.7500000000000000000 ) ) ;
#18017=ORIENTED_EDGE ( 'NONE', *, *, #29169, .F. ) ;
#18019=CARTESIAN_POINT ( 'NONE',  ( -6.500000000000000000, 0.000000000000000000, 3.180000000000000160 ) ) ;
#18063=ORIENTED_EDGE ( 'NONE', *, *, #35049, .T. ) ;
#18077=EDGE_CURVE ( 'NONE', #2729, #22127, #8774, .T. ) ;
#18097=CARTESIAN_POINT ( 'NONE',  ( -6.500000000000000000, 0.000000000000000000, -0.7520000000000004459 ) ) ;
#18135=LINE ( 'NONE', #2084, #7792 ) ;
#18149=LINE ( 'NONE', #7071, #28806 ) ;
#18181=DIRECTION ( 'NONE',  ( -1.000000000000000000, 0.000000000000000000, 0.000000000000000000 ) ) ;
#18204=CARTESIAN_POINT ( 'NONE',  ( 10.00000000000000000, -1.505030548027689319, 3.180000000000000160 ) ) ;
#18241=AXIS2_PLACEMENT_3D ( 'NONE', #25772, #6553, #31129 ) ;
#18255=DIRECTION ( 'NONE',  ( 1.000000000000000000, 0.000000000000000000, 0.000000000000000000 ) ) ;
#18267=ORIENTED_EDGE ( 'NONE', *, *, #31144, .F. ) ;
#18301=DIRECTION ( 'NONE',  ( 0.000000000000000000, 0.000000000000000000, -1.000000000000000000 ) ) ;
#18370=DIRECTION ( 'NONE',  ( -1.000000000000000000, 0.000000000000000000, -0.000000000000000000 ) ) ;
#18372=FACE_OUTER_BOUND ( 'NONE', #12171, .T. ) ;
#18387=CARTESIAN_POINT ( 'NONE',  ( 0.000000000000000000, 0.000000000000000000, -0.7500000000000000000 ) ) ;
#18417=VERTEX_POINT ( 'NONE', #14090 ) ;
#18418=CIRCLE ( 'NONE', #12168, 4.306175033202026547 ) ;
#18439=UNCERTAINTY_MEASURE_WITH_UNIT (LENGTH_MEASURE( 1.000000000000000082E-05 ), #22430, 'distance_accuracy_value', 'NONE');
#18521=EDGE_LOOP ( 'NONE', ( #20096, #9365, #26954, #24804 ) ) ;
#18522=CIRCLE ( 'NONE', #3143, 1.649999999999999467 ) ;
#18665=EDGE_CURVE ( 'NONE', #29588, #22009, #23082, .T. ) ;
#18767=FACE_BOUND ( 'NONE', #11145, .T. ) ;
#18770=EDGE_LOOP ( 'NONE', ( #10115, #10926, #2394, #11156 ) ) ;
#18796=VERTEX_POINT ( 'NONE', #26999 ) ;
#18807=ORIENTED_EDGE ( 'NONE', *, *, #35049, .F. ) ;
#18820=FACE_OUTER_BOUND ( 'NONE', #24536, .T. ) ;
#18881=CARTESIAN_POINT ( 'NONE',  ( -5.344999999999999751, 1.414467053015192657E-16, 3.930000000000000160 ) ) ;
#18913=DIRECTION ( 'NONE',  ( -1.000000000000000000, 8.881784197001254296E-16, 0.000000000000000000 ) ) ;
#19054=EDGE_LOOP ( 'NONE', ( #24677, #19739, #6791, #4951, #9049 ) ) ;
#19124=VECTOR ( 'NONE', #27969, 1000.000000000000000 ) ;
#19192=DIRECTION ( 'NONE',  ( -0.000000000000000000, -0.000000000000000000, -1.000000000000000000 ) ) ;
#19215=VECTOR ( 'NONE', #27442, 1000.000000000000000 ) ;
#19271=DIRECTION ( 'NONE',  ( -1.000000000000000000, 0.000000000000000000, 0.000000000000000000 ) ) ;
#19350=DIRECTION ( 'NONE',  ( -0.000000000000000000, -0.000000000000000000, -1.000000000000000000 ) ) ;
#19400=CARTESIAN_POINT ( 'NONE',  ( -3.250000000000000000, -5.838643359331793015, 3.930000000000000160 ) ) ;
#19428=CIRCLE ( 'NONE', #2914, 1.649999999999999467 ) ;
#19438=EDGE_LOOP ( 'NONE', ( #14847, #13465, #26234, #13774 ) ) ;
#19491=ADVANCED_FACE ( 'NONE', ( #1649 ), #25861, .T. ) ;
#19492=DIRECTION ( 'NONE',  ( -0.000000000000000000, -0.000000000000000000, -1.000000000000000000 ) ) ;
#19585=VECTOR ( 'NONE', #12023, 1000.000000000000000 ) ;
#19650=EDGE_LOOP ( 'NONE', ( #24571, #30132 ) ) ;
#19656=EDGE_CURVE ( 'NONE', #33286, #24787, #24401, .T. ) ;
#19709=FACE_OUTER_BOUND ( 'NONE', #23094, .T. ) ;
#19712=ORIENTED_EDGE ( 'NONE', *, *, #27631, .T. ) ;
#19723=CIRCLE ( 'NONE', #6045, 1.155000000000000027 ) ;
#19739=ORIENTED_EDGE ( 'NONE', *, *, #26484, .F. ) ;
#19790=AXIS2_PLACEMENT_3D ( 'NONE', #18387, #26028, #12872 ) ;
#19805=ORIENTED_EDGE ( 'NONE', *, *, #31144, .T. ) ;
#19824=ORIENTED_EDGE ( 'NONE', *, *, #18665, .F. ) ;
#19864=FACE_OUTER_BOUND ( 'NONE', #25467, .T. ) ;
#19905=LINE ( 'NONE', #26405, #5798 ) ;
#19990=EDGE_CURVE ( 'NONE', #21780, #17552, #22804, .T. ) ;
#20070=ORIENTED_EDGE ( 'NONE', *, *, #20136, .T. ) ;
#20083=VECTOR ( 'NONE', #1494, 1000.000000000000000 ) ;
#20096=ORIENTED_EDGE ( 'NONE', *, *, #26747, .F. ) ;
#20136=EDGE_CURVE ( 'NONE', #8625, #3609, #19723, .T. ) ;
#20283=VECTOR ( 'NONE', #22455, 1000.000000000000000 ) ;
#20422=CIRCLE ( 'NONE', #11352, 1.649999999999999467 ) ;
#20434=CYLINDRICAL_SURFACE ( 'NONE', #4172, 4.306175033202026547 ) ;
#20453=VERTEX_POINT ( 'NONE', #32166 ) ;
#20454=EDGE_CURVE ( 'NONE', #22009, #3503, #18149, .T. ) ;
#20499=CARTESIAN_POINT ( 'NONE',  ( -4.875000000000000000, 2.702098422956710877, -0.7500000000000000000 ) ) ;
#20504=ORIENTED_EDGE ( 'NONE', *, *, #7802, .T. ) ;
#20561=FACE_OUTER_BOUND ( 'NONE', #22670, .T. ) ;
#20583=AXIS2_PLACEMENT_3D ( 'NONE', #8832, #33393, #12232 ) ;
#20632=DIRECTION ( 'NONE',  ( 0.000000000000000000, 0.000000000000000000, 1.000000000000000000 ) ) ;
#20719=AXIS2_PLACEMENT_3D ( 'NONE', #10382, #10915, #24951 ) ;
#20777=DIRECTION ( 'NONE',  ( 1.000000000000000000, 0.000000000000000000, 0.000000000000000000 ) ) ;
#20829=CARTESIAN_POINT ( 'NONE',  ( 0.000000000000000000, 0.000000000000000000, -0.7500000000000000000 ) ) ;
#20830=EDGE_LOOP ( 'NONE', ( #4826, #31675, #7141, #31841, #22064 ) ) ;
#20850=( LENGTH_UNIT ( ) NAMED_UNIT ( * ) SI_UNIT ( .MILLI., .METRE. ) );
#20910=VERTEX_POINT ( 'NONE', #29417 ) ;
#20914=DIRECTION ( 'NONE',  ( -0.000000000000000000, -0.000000000000000000, -1.000000000000000000 ) ) ;
#20989=ORIENTED_EDGE ( 'NONE', *, *, #18077, .F. ) ;
#21015=DIRECTION ( 'NONE',  ( 1.000000000000000000, 0.000000000000000000, 0.000000000000000000 ) ) ;
#21016=DIRECTION ( 'NONE',  ( 1.000000000000000000, 0.000000000000000000, 0.000000000000000000 ) ) ;
#21022=LINE ( 'NONE', #15883, #14867 ) ;
#21045=LINE ( 'NONE', #23883, #15428 ) ;
#21049=EDGE_CURVE ( 'NONE', #3348, #18796, #16786, .T. ) ;
#21367=CARTESIAN_POINT ( 'NONE',  ( -1.649999999999999911, 0.000000000000000000, 3.180000000000000160 ) ) ;
#21369=AXIS2_PLACEMENT_3D ( 'NONE', #15367, #17354, #3789 ) ;
#21453=CARTESIAN_POINT ( 'NONE',  ( -8.149999999999998579, 2.020667218593133001E-16, 0.000000000000000000 ) ) ;
#21466=CIRCLE ( 'NONE', #34517, 1.999999999999999556 ) ;
#21496=CARTESIAN_POINT ( 'NONE',  ( -1.625000000000000000, 2.702098422956710877, 3.930000000000000160 ) ) ;
#21510=EDGE_CURVE ( 'NONE', #16280, #33055, #4416, .T. ) ;
#21564=ADVANCED_BREP_SHAPE_REPRESENTATION ( '', ( #827, #28566 ), #6416 ) ;
#21565=DIRECTION ( 'NONE',  ( 0.000000000000000000, 0.000000000000000000, -1.000000000000000000 ) ) ;
#21705=DIRECTION ( 'NONE',  ( -0.000000000000000000, -0.000000000000000000, -1.000000000000000000 ) ) ;
#21720=DIRECTION ( 'NONE',  ( -0.000000000000000000, -0.000000000000000000, 1.000000000000000000 ) ) ;
#21729=CARTESIAN_POINT ( 'NONE',  ( -6.500000000000000000, 0.000000000000000000, -0.7500000000000000000 ) ) ;
#21741=DIRECTION ( 'NONE',  ( -0.000000000000000000, -0.000000000000000000, -1.000000000000000000 ) ) ;
#21780=VERTEX_POINT ( 'NONE', #18881 ) ;
#21800=ORIENTED_EDGE ( 'NONE', *, *, #15235, .T. ) ;
#21805=VERTEX_POINT ( 'NONE', #13885 ) ;
#21836=VERTEX_POINT ( 'NONE', #2302 ) ;
#21853=EDGE_CURVE ( 'NONE', #24787, #1716, #30534, .T. ) ;
#21881=DIRECTION ( 'NONE',  ( 1.000000000000000000, 0.000000000000000000, 0.000000000000000000 ) ) ;
#21882=DIRECTION ( 'NONE',  ( 1.000000000000000000, 0.000000000000000000, 0.000000000000000000 ) ) ;
#21898=EDGE_CURVE ( 'NONE', #21805, #18796, #15192, .T. ) ;
#21909=CLOSED_SHELL ( 'NONE', ( #24742, #2774, #24777, #32077, #19491, #5440, #14573, #24557, #24947, #5770, #17238, #34467, #24812, #15935, #23672, #3515, #26767, #12433, #22683, #25541, #12588, #1454, #15933, #9640, #26585, #13828 ) ) ;
#21920=FACE_OUTER_BOUND ( 'NONE', #30245, .T. ) ;
#21926=CARTESIAN_POINT ( 'NONE',  ( -5.527271473480783293, -1.747512292859696226, -0.7500000000000000000 ) ) ;
#21955=ORIENTED_EDGE ( 'NONE', *, *, #15053, .T. ) ;
#21989=FACE_OUTER_BOUND ( 'NONE', #20830, .T. ) ;
#22009=VERTEX_POINT ( 'NONE', #21453 ) ;
#22064=ORIENTED_EDGE ( 'NONE', *, *, #14015, .T. ) ;
#22076=( NAMED_UNIT ( * ) SI_UNIT ( $, .STERADIAN. ) SOLID_ANGLE_UNIT ( ) );
#22127=VERTEX_POINT ( 'NONE', #88 ) ;
#22172=EDGE_CURVE ( 'NONE', #7199, #199, #27304, .T. ) ;
#22310=CARTESIAN_POINT ( 'NONE',  ( -3.250000000000000000, 5.404196845913421754, 0.000000000000000000 ) ) ;
#22342=CARTESIAN_POINT ( 'NONE',  ( -6.500000000000000000, 0.000000000000000000, 3.930000000000000160 ) ) ;
#22430=( LENGTH_UNIT ( ) NAMED_UNIT ( * ) SI_UNIT ( .MILLI., .METRE. ) );
#22455=DIRECTION ( 'NONE',  ( -0.000000000000000000, -0.000000000000000000, -1.000000000000000000 ) ) ;
#22512=LINE ( 'NONE', #27661, #31085 ) ;
#22602=DIRECTION ( 'NONE',  ( -0.000000000000000000, -0.000000000000000000, -1.000000000000000000 ) ) ;
#22629=DIRECTION ( 'NONE',  ( -1.000000000000000000, 0.000000000000000000, 0.000000000000000000 ) ) ;
#22646=EDGE_CURVE ( 'NONE', #33401, #3348, #31332, .T. ) ;
#22661=AXIS2_PLACEMENT_3D ( 'NONE', #19400, #21705, #21881 ) ;
#22670=EDGE_LOOP ( 'NONE', ( #18807, #20504, #34811, #33675 ) ) ;
#22673=EDGE_CURVE ( 'NONE', #10814, #24787, #34774, .T. ) ;
#22683=ADVANCED_FACE ( 'NONE', ( #23685 ), #28846, .T. ) ;
#22694=CARTESIAN_POINT ( 'NONE',  ( -5.469264258321805627, 1.713938105891546382, 3.930000000000000160 ) ) ;
#22728=CARTESIAN_POINT ( 'NONE',  ( -6.500000000000000000, 0.000000000000000000, -0.7500000000000000000 ) ) ;
#22804=LINE ( 'NONE', #4599, #17459 ) ;
#22814=DIRECTION ( 'NONE',  ( -1.000000000000000000, 0.000000000000000000, 0.000000000000000000 ) ) ;
#22862=CARTESIAN_POINT ( 'NONE',  ( 0.000000000000000000, 0.000000000000000000, 0.000000000000000000 ) ) ;
#22872=FACE_OUTER_BOUND ( 'NONE', #8918, .T. ) ;
#22897=DIRECTION ( 'NONE',  ( 1.000000000000000000, 0.000000000000000000, 0.000000000000000000 ) ) ;
#22917=CARTESIAN_POINT ( 'NONE',  ( -1.030735741678193262, 1.713938105891546382, 3.930000000000000160 ) ) ;
#23082=CIRCLE ( 'NONE', #7708, 1.649999999999999467 ) ;
#23094=EDGE_LOOP ( 'NONE', ( #2602, #33995, #24310, #20070 ) ) ;
#23097=STYLED_ITEM('',(#35289),#827);
#23165=VERTEX_POINT ( 'NONE', #8321 ) ;
#23176=PLANE ( 'NONE',  #34714 ) ;
#23321=AXIS2_PLACEMENT_3D ( 'NONE', #21729, #29925, #5519 ) ;
#23534=ORIENTED_EDGE ( 'NONE', *, *, #14015, .F. ) ;
#23605=DIRECTION ( 'NONE',  ( 1.000000000000000000, 0.000000000000000000, 0.000000000000000000 ) ) ;
#23625=EDGE_CURVE ( 'NONE', #12505, #7313, #6929, .T. ) ;
#23630=VERTEX_POINT ( 'NONE', #33854 ) ;
#23643=DIRECTION ( 'NONE',  ( 1.000000000000000000, 0.000000000000000000, 0.000000000000000000 ) ) ;
#23655=ORIENTED_EDGE ( 'NONE', *, *, #34274, .T. ) ;
#23672=ADVANCED_FACE ( 'NONE', ( #24637, #28510, #21989 ), #23176, .T. ) ;
#23676=AXIS2_PLACEMENT_3D ( 'NONE', #32988, #33175, #11478 ) ;
#23685=FACE_OUTER_BOUND ( 'NONE', #16316, .T. ) ;
#23727=ORIENTED_EDGE ( 'NONE', *, *, #4398, .T. ) ;
#23740=EDGE_CURVE ( 'NONE', #9411, #2729, #21022, .T. ) ;
#23744=DIRECTION ( 'NONE',  ( -0.000000000000000000, -0.000000000000000000, 1.000000000000000000 ) ) ;
#23756=VECTOR ( 'NONE', #33347, 1000.000000000000000 ) ;
#23883=CARTESIAN_POINT ( 'NONE',  ( 10.00000000000000000, -1.505030548027689319, 3.180000000000000160 ) ) ;
#23978=AXIS2_PLACEMENT_3D ( 'NONE', #26305, #29514, #23643 ) ;
#24055=ORIENTED_EDGE ( 'NONE', *, *, #4235, .T. ) ;
#24117=ORIENTED_EDGE ( 'NONE', *, *, #25456, .F. ) ;
#24201=VECTOR ( 'NONE', #5931, 1000.000000000000000 ) ;
#24216=PRODUCT_DEFINITION_CONTEXT ( 'detailed design', #33968, 'design' ) ;
#24227=FACE_BOUND ( 'NONE', #28322, .T. ) ;
#24264=AXIS2_PLACEMENT_3D ( 'NONE', #3579, #14466, #25298 ) ;
#24296=EDGE_CURVE ( 'NONE', #9411, #18417, #2938, .T. ) ;
#24299=CYLINDRICAL_SURFACE ( 'NONE', #7797, 1.649999999999999467 ) ;
#24308=CYLINDRICAL_SURFACE ( 'NONE', #17679, 1.649999999999999911 ) ;
#24310=ORIENTED_EDGE ( 'NONE', *, *, #2472, .T. ) ;
#24401=LINE ( 'NONE', #6058, #20283 ) ;
#24442=LINE ( 'NONE', #32815, #24201 ) ;
#24484=FACE_OUTER_BOUND ( 'NONE', #26610, .T. ) ;
#24536=EDGE_LOOP ( 'NONE', ( #1527, #25268, #33699, #17726 ) ) ;
#24557=ADVANCED_FACE ( 'NONE', ( #15434 ), #26272, .T. ) ;
#24568=CYLINDRICAL_SURFACE ( 'NONE', #13901, 1.649999999999999467 ) ;
#24569=CARTESIAN_POINT ( 'NONE',  ( -8.149999999999998579, 2.020667218593133001E-16, 3.180000000000000160 ) ) ;
#24571=ORIENTED_EDGE ( 'NONE', *, *, #20136, .F. ) ;
#24588=CARTESIAN_POINT ( 'NONE',  ( -5.823698994896891357, -1.505030548027689319, 3.180000000000000160 ) ) ;
#24637=FACE_BOUND ( 'NONE', #25050, .T. ) ;
#24660=EDGE_LOOP ( 'NONE', ( #21800, #168, #14602, #7764 ) ) ;
#24677=ORIENTED_EDGE ( 'NONE', *, *, #4398, .F. ) ;
#24742=ADVANCED_FACE ( 'NONE', ( #19864 ), #33369, .F. ) ;
#24777=ADVANCED_FACE ( 'NONE', ( #24826 ), #11489, .T. ) ;
#24787=VERTEX_POINT ( 'NONE', #7780 ) ;
#24804=ORIENTED_EDGE ( 'NONE', *, *, #32135, .T. ) ;
#24812=ADVANCED_FACE ( 'NONE', ( #28980 ), #4749, .F. ) ;
#24826=FACE_OUTER_BOUND ( 'NONE', #33082, .T. ) ;
#24912=ORIENTED_EDGE ( 'NONE', *, *, #19656, .F. ) ;
#24925=CARTESIAN_POINT ( 'NONE',  ( 0.6763010051031069780, -1.505030548027689319, 3.180000000000000160 ) ) ;
#24930=CARTESIAN_POINT ( 'NONE',  ( 0.000000000000000000, 0.000000000000000000, 3.180000000000000160 ) ) ;
#24947=ADVANCED_FACE ( 'NONE', ( #5460 ), #314, .T. ) ;
#24951=DIRECTION ( 'NONE',  ( 1.000000000000000000, 0.000000000000000000, 0.000000000000000000 ) ) ;
#24985=CARTESIAN_POINT ( 'NONE',  ( -1.030735741678193262, 1.713938105891546382, 3.930000000000000160 ) ) ;
#24993=DIRECTION ( 'NONE',  ( -0.000000000000000000, -0.000000000000000000, -1.000000000000000000 ) ) ;
#25050=EDGE_LOOP ( 'NONE', ( #15831, #34643 ) ) ;
#25066=DIRECTION ( 'NONE',  ( 1.000000000000000000, 0.000000000000000000, 0.000000000000000000 ) ) ;
#25140=AXIS2_PLACEMENT_3D ( 'NONE', #1198, #12076, #33770 ) ;
#25158=DIRECTION ( 'NONE',  ( -1.000000000000000000, 0.000000000000000000, 0.000000000000000000 ) ) ;
#25196=DIRECTION ( 'NONE',  ( -1.000000000000000000, 0.000000000000000000, 0.000000000000000000 ) ) ;
#25216=DIRECTION ( 'NONE',  ( -0.000000000000000000, -0.000000000000000000, 1.000000000000000000 ) ) ;
#25223=AXIS2_PLACEMENT_3D ( 'NONE', #33716, #12203, #15044 ) ;
#25268=ORIENTED_EDGE ( 'NONE', *, *, #26747, .T. ) ;
#25298=DIRECTION ( 'NONE',  ( 1.000000000000000000, 0.000000000000000000, 0.000000000000000000 ) ) ;
#25337=VERTEX_POINT ( 'NONE', #15251 ) ;
#25456=EDGE_CURVE ( 'NONE', #30822, #20910, #29815, .T. ) ;
#25467=EDGE_LOOP ( 'NONE', ( #27501, #13975, #26841, #1066 ) ) ;
#25521=LINE ( 'NONE', #9515, #31013 ) ;
#25541=ADVANCED_FACE ( 'NONE', ( #4146 ), #1325, .F. ) ;
#25544=CARTESIAN_POINT ( 'NONE',  ( 0.000000000000000000, 0.000000000000000000, 3.931000000000000494 ) ) ;
#25570=CYLINDRICAL_SURFACE ( 'NONE', #25140, 1.999999999999999556 ) ;
#25644=ORIENTED_EDGE ( 'NONE', *, *, #19990, .F. ) ;
#25647=DIRECTION ( 'NONE',  ( 0.000000000000000000, 0.000000000000000000, -1.000000000000000000 ) ) ;
#25772=CARTESIAN_POINT ( 'NONE',  ( -3.250000000000000000, -5.838643359331793015, -0.7500000000000000000 ) ) ;
#25783=DIRECTION ( 'NONE',  ( -0.000000000000000000, -0.000000000000000000, 1.000000000000000000 ) ) ;
#25861=CYLINDRICAL_SURFACE ( 'NONE', #21369, 1.649999999999999467 ) ;
#25877=CARTESIAN_POINT ( 'NONE',  ( -1.155000000000000027, 0.000000000000000000, -0.7500000000000000000 ) ) ;
#25988=EDGE_LOOP ( 'NONE', ( #25644, #18017, #35074, #14445 ) ) ;
#26007=CIRCLE ( 'NONE', #991, 1.154999999999999805 ) ;
#26028=DIRECTION ( 'NONE',  ( 0.000000000000000000, 0.000000000000000000, -1.000000000000000000 ) ) ;
#26049=EDGE_CURVE ( 'NONE', #35075, #30822, #18418, .T. ) ;
#26234=ORIENTED_EDGE ( 'NONE', *, *, #28802, .F. ) ;
#26272=CYLINDRICAL_SURFACE ( 'NONE', #29092, 1.649999999999999911 ) ;
#26305=CARTESIAN_POINT ( 'NONE',  ( -3.250000000000000000, -5.838643359331793015, -0.7500000000000000000 ) ) ;
#26336=DIRECTION ( 'NONE',  ( 0.000000000000000000, 0.000000000000000000, -1.000000000000000000 ) ) ;
#26378=ORIENTED_EDGE ( 'NONE', *, *, #6899, .F. ) ;
#26405=CARTESIAN_POINT ( 'NONE',  ( -4.850000000000000533, 0.000000000000000000, -0.7520000000000004459 ) ) ;
#26484=EDGE_CURVE ( 'NONE', #1716, #4705, #12752, .T. ) ;
#26491=ORIENTED_EDGE ( 'NONE', *, *, #22673, .T. ) ;
#26509=DIRECTION ( 'NONE',  ( 0.000000000000000000, 0.000000000000000000, -1.000000000000000000 ) ) ;
#26579=CARTESIAN_POINT ( 'NONE',  ( 0.000000000000000000, 0.000000000000000000, 0.000000000000000000 ) ) ;
#26585=ADVANCED_FACE ( 'NONE', ( #32349 ), #29688, .T. ) ;
#26610=EDGE_LOOP ( 'NONE', ( #33426, #14444, #771, #3812, #3254 ) ) ;
#26672=CIRCLE ( 'NONE', #34070, 1.999999999999999556 ) ;
#26747=EDGE_CURVE ( 'NONE', #2399, #20453, #30703, .T. ) ;
#26767=ADVANCED_FACE ( 'NONE', ( #22872 ), #14345, .T. ) ;
#26769=DIRECTION ( 'NONE',  ( -0.000000000000000000, -0.000000000000000000, -1.000000000000000000 ) ) ;
#26795=CARTESIAN_POINT ( 'NONE',  ( 0.000000000000000000, 0.000000000000000000, 0.000000000000000000 ) ) ;
#26825=DIRECTION ( 'NONE',  ( -0.000000000000000000, -0.000000000000000000, 1.000000000000000000 ) ) ;
#26835=EDGE_CURVE ( 'NONE', #2399, #29809, #33803, .T. ) ;
#26841=ORIENTED_EDGE ( 'NONE', *, *, #8995, .T. ) ;
#26920=CARTESIAN_POINT ( 'NONE',  ( -7.176301005103106867, -1.505030548027689319, 0.000000000000000000 ) ) ;
#26954=ORIENTED_EDGE ( 'NONE', *, *, #3446, .F. ) ;
#26999=CARTESIAN_POINT ( 'NONE',  ( -0.9727285265192152641, -1.747512292859696670, 0.000000000000000000 ) ) ;
#27036=EDGE_LOOP ( 'NONE', ( #7492, #989, #11591, #4120 ) ) ;
#27055=CARTESIAN_POINT ( 'NONE',  ( 1.999999999999999556, 0.000000000000000000, -0.7500000000000000000 ) ) ;
#27130=CARTESIAN_POINT ( 'NONE',  ( -5.823698994896891357, -1.505030548027689319, 0.000000000000000000 ) ) ;
#27136=DIRECTION ( 'NONE',  ( -0.000000000000000000, -0.000000000000000000, -1.000000000000000000 ) ) ;
#27259=DIRECTION ( 'NONE',  ( -0.000000000000000000, -0.000000000000000000, 1.000000000000000000 ) ) ;
#27304=LINE ( 'NONE', #14863, #20083 ) ;
#27324=DIRECTION ( 'NONE',  ( -0.000000000000000000, -0.000000000000000000, 1.000000000000000000 ) ) ;
#27431=PLANE ( 'NONE',  #34593 ) ;
#27442=DIRECTION ( 'NONE',  ( -0.000000000000000000, -0.000000000000000000, 1.000000000000000000 ) ) ;
#27501=ORIENTED_EDGE ( 'NONE', *, *, #15053, .F. ) ;
#27631=EDGE_CURVE ( 'NONE', #18417, #22127, #9949, .T. ) ;
#27661=CARTESIAN_POINT ( 'NONE',  ( -8.499999999999998224, 0.000000000000000000, 3.930000000000000160 ) ) ;
#27681=DIRECTION ( 'NONE',  ( 1.000000000000000000, 0.000000000000000000, 0.000000000000000000 ) ) ;
#27746=DIRECTION ( 'NONE',  ( -0.000000000000000000, -0.000000000000000000, -1.000000000000000000 ) ) ;
#27749=CARTESIAN_POINT ( 'NONE',  ( -3.250000000000000000, -5.838643359331793015, 3.180000000000000160 ) ) ;
#27765=AXIS2_PLACEMENT_3D ( 'NONE', #14943, #21741, #19271 ) ;
#27788=ORIENTED_EDGE ( 'NONE', *, *, #4767, .T. ) ;
#27891=CARTESIAN_POINT ( 'NONE',  ( 0.6763010051031080883, -1.505030548027688875, 0.000000000000000000 ) ) ;
#27913=AXIS2_PLACEMENT_3D ( 'NONE', #32107, #26769, #13261 ) ;
#27961=VERTEX_POINT ( 'NONE', #27891 ) ;
#27969=DIRECTION ( 'NONE',  ( -0.000000000000000000, -0.000000000000000000, -1.000000000000000000 ) ) ;
#28033=AXIS2_PLACEMENT_3D ( 'NONE', #33180, #3972, #9332 ) ;
#28037=VERTEX_POINT ( 'NONE', #1888 ) ;
#28039=ORIENTED_EDGE ( 'NONE', *, *, #27631, .F. ) ;
#28107=EDGE_LOOP ( 'NONE', ( #3951, #33681, #31167, #2580 ) ) ;
#28231=SHAPE_REPRESENTATION ( 'chainlinkage', ( #28566 ), #6416 ) ;
#28250=AXIS2_PLACEMENT_3D ( 'NONE', #9104, #14464, #8748 ) ;
#28322=EDGE_LOOP ( 'NONE', ( #12658, #17078, #26378, #19824 ) ) ;
#28333=CARTESIAN_POINT ( 'NONE',  ( 0.000000000000000000, 0.000000000000000000, 3.930000000000000160 ) ) ;
#28384=DIRECTION ( 'NONE',  ( 1.000000000000000000, 0.000000000000000000, 0.000000000000000000 ) ) ;
#28408=CARTESIAN_POINT ( 'NONE',  ( -0.6763010051031078662, -1.505030548027689319, 0.000000000000000000 ) ) ;
#28510=FACE_BOUND ( 'NONE', #19650, .T. ) ;
#28547=AXIS2_PLACEMENT_3D ( 'NONE', #30165, #24993, #6300 ) ;
#28566=AXIS2_PLACEMENT_3D ( 'NONE', #26579, #2200, #13073 ) ;
#28693=ORIENTED_EDGE ( 'NONE', *, *, #21853, .T. ) ;
#28802=EDGE_CURVE ( 'NONE', #3348, #33660, #16536, .T. ) ;
#28806=VECTOR ( 'NONE', #26825, 1000.000000000000000 ) ;
#28813=AXIS2_PLACEMENT_3D ( 'NONE', #7404, #18301, #14364 ) ;
#28818=EDGE_LOOP ( 'NONE', ( #6733, #21955 ) ) ;
#28846=CYLINDRICAL_SURFACE ( 'NONE', #4059, 1.999999999999999112 ) ;
#28870=AXIS2_PLACEMENT_3D ( 'NONE', #14006, #19350, #17045 ) ;
#28895=VECTOR ( 'NONE', #2860, 1000.000000000000000 ) ;
#28961=DIRECTION ( 'NONE',  ( -0.000000000000000000, -0.000000000000000000, -1.000000000000000000 ) ) ;
#28980=FACE_OUTER_BOUND ( 'NONE', #19438, .T. ) ;
#29092=AXIS2_PLACEMENT_3D ( 'NONE', #2069, #14916, #1377 ) ;
#29161=CARTESIAN_POINT ( 'NONE',  ( 0.000000000000000000, 0.000000000000000000, 3.180000000000000160 ) ) ;
#29169=EDGE_CURVE ( 'NONE', #12730, #21780, #55, .T. ) ;
#29186=CARTESIAN_POINT ( 'NONE',  ( -6.500000000000000000, 0.000000000000000000, -0.7500000000000000000 ) ) ;
#29213=DIRECTION ( 'NONE',  ( 1.000000000000000000, 0.000000000000000000, 0.000000000000000000 ) ) ;
#29254=VERTEX_POINT ( 'NONE', #2344 ) ;
#29323=VERTEX_POINT ( 'NONE', #31885 ) ;
#29356=CIRCLE ( 'NONE', #14016, 1.649999999999999911 ) ;
#29417=CARTESIAN_POINT ( 'NONE',  ( -5.469264258321805627, 1.713938105891546382, 3.180000000000000160 ) ) ;
#29514=DIRECTION ( 'NONE',  ( -0.000000000000000000, -0.000000000000000000, 1.000000000000000000 ) ) ;
#29588=VERTEX_POINT ( 'NONE', #9799 ) ;
#29636=EDGE_LOOP ( 'NONE', ( #34975, #5340, #18267, #24055 ) ) ;
#29688=PLANE ( 'NONE',  #30927 ) ;
#29730=DIRECTION ( 'NONE',  ( 1.000000000000000000, 0.000000000000000000, 0.000000000000000000 ) ) ;
#29809=VERTEX_POINT ( 'NONE', #21367 ) ;
#29815=LINE ( 'NONE', #16307, #30879 ) ;
#29913=CARTESIAN_POINT ( 'NONE',  ( -6.500000000000000000, 0.000000000000000000, 3.930000000000000160 ) ) ;
#29925=DIRECTION ( 'NONE',  ( 0.000000000000000000, 0.000000000000000000, -1.000000000000000000 ) ) ;
#29927=EDGE_CURVE ( 'NONE', #3503, #16280, #19428, .T. ) ;
#29944=CARTESIAN_POINT ( 'NONE',  ( -0.9727285265192152641, -1.747512292859696670, -0.7500000000000000000 ) ) ;
#29947=PRODUCT_DEFINITION_SHAPE ( 'NONE', 'NONE',  #32294 ) ;
#30080=DIRECTION ( 'NONE',  ( 0.000000000000000000, 0.000000000000000000, -1.000000000000000000 ) ) ;
#30094=ORIENTED_EDGE ( 'NONE', *, *, #26049, .F. ) ;
#30098=PRODUCT_CONTEXT ( 'NONE', #10309, 'mechanical' ) ;
#30101=CARTESIAN_POINT ( 'NONE',  ( -8.499999999999998224, 0.000000000000000000, 3.180000000000000160 ) ) ;
#30124=DIRECTION ( 'NONE',  ( -0.000000000000000000, -0.000000000000000000, -1.000000000000000000 ) ) ;
#30127=AXIS2_PLACEMENT_3D ( 'NONE', #18204, #5167, #21565 ) ;
#30132=ORIENTED_EDGE ( 'NONE', *, *, #3324, .F. ) ;
#30157=AXIS2_PLACEMENT_3D ( 'NONE', #11810, #12154, #31185 ) ;
#30165=CARTESIAN_POINT ( 'NONE',  ( -6.500000000000000000, 0.000000000000000000, 3.931000000000000494 ) ) ;
#30219=EDGE_LOOP ( 'NONE', ( #10090, #7936, #19805, #4664 ) ) ;
#30245=EDGE_LOOP ( 'NONE', ( #20989, #34248, #15433, #14096, #13595 ) ) ;
#30382=CARTESIAN_POINT ( 'NONE',  ( 0.000000000000000000, 0.000000000000000000, 3.180000000000000160 ) ) ;
#30466=DIRECTION ( 'NONE',  ( 0.000000000000000000, 0.000000000000000000, 1.000000000000000000 ) ) ;
#30499=DIRECTION ( 'NONE',  ( -1.000000000000000000, 0.000000000000000000, 0.000000000000000000 ) ) ;
#30517=CARTESIAN_POINT ( 'NONE',  ( 0.000000000000000000, 0.000000000000000000, 0.000000000000000000 ) ) ;
#30534=CIRCLE ( 'NONE', #2676, 4.682234377621698584 ) ;
#30557=FACE_OUTER_BOUND ( 'NONE', #34102, .T. ) ;
#30703=LINE ( 'NONE', #1503, #19585 ) ;
#30822=VERTEX_POINT ( 'NONE', #22694 ) ;
#30854=LINE ( 'NONE', #16830, #23756 ) ;
#30868=EDGE_CURVE ( 'NONE', #20453, #21836, #10931, .T. ) ;
#30879=VECTOR ( 'NONE', #27136, 1000.000000000000000 ) ;
#30893=DIRECTION ( 'NONE',  ( -0.000000000000000000, -0.000000000000000000, -1.000000000000000000 ) ) ;
#30927=AXIS2_PLACEMENT_3D ( 'NONE', #13496, #8322, #138 ) ;
#30956=CARTESIAN_POINT ( 'NONE',  ( 0.000000000000000000, 0.000000000000000000, 0.000000000000000000 ) ) ;
#30961=LINE ( 'NONE', #6740, #12412 ) ;
#31013=VECTOR ( 'NONE', #12016, 1000.000000000000000 ) ;
#31063=CIRCLE ( 'NONE', #15726, 1.649999999999999911 ) ;
#31085=VECTOR ( 'NONE', #19492, 1000.000000000000000 ) ;
#31129=DIRECTION ( 'NONE',  ( 1.000000000000000000, 0.000000000000000000, 0.000000000000000000 ) ) ;
#31144=EDGE_CURVE ( 'NONE', #29254, #199, #710, .T. ) ;
#31152=VECTOR ( 'NONE', #5331, 1000.000000000000000 ) ;
#31167=ORIENTED_EDGE ( 'NONE', *, *, #21510, .F. ) ;
#31182=DIRECTION ( 'NONE',  ( 0.000000000000000000, 0.000000000000000000, 1.000000000000000000 ) ) ;
#31185=DIRECTION ( 'NONE',  ( 1.000000000000000000, 0.000000000000000000, 0.000000000000000000 ) ) ;
#31332=CIRCLE ( 'NONE', #16009, 1.999999999999999556 ) ;
#31362=EDGE_LOOP ( 'NONE', ( #28693, #34454, #4673, #17640 ) ) ;
#31398=DIRECTION ( 'NONE',  ( 0.000000000000000000, 0.000000000000000000, 1.000000000000000000 ) ) ;
#31438=EDGE_LOOP ( 'NONE', ( #14116, #16308, #11843, #31916 ) ) ;
#31624=CARTESIAN_POINT ( 'NONE',  ( -3.250000000000000000, 5.404196845913421754, -0.7500000000000000000 ) ) ;
#31639=CARTESIAN_POINT ( 'NONE',  ( 1.155000000000000027, 1.414467053015192904E-16, 3.931000000000000494 ) ) ;
#31675=ORIENTED_EDGE ( 'NONE', *, *, #2514, .T. ) ;
#31698=ORIENTED_EDGE ( 'NONE', *, *, #23740, .T. ) ;
#31841=ORIENTED_EDGE ( 'NONE', *, *, #28802, .T. ) ;
#31851=DIRECTION ( 'NONE',  ( -0.000000000000000000, -0.000000000000000000, -1.000000000000000000 ) ) ;
#31877=CARTESIAN_POINT ( 'NONE',  ( -0.6763010051031069780, -1.505030548027689319, 3.180000000000000160 ) ) ;
#31885=CARTESIAN_POINT ( 'NONE',  ( -5.527271473480783293, -1.747512292859696226, 0.000000000000000000 ) ) ;
#31916=ORIENTED_EDGE ( 'NONE', *, *, #21049, .F. ) ;
#32077=ADVANCED_FACE ( 'NONE', ( #34425 ), #25570, .T. ) ;
#32107=CARTESIAN_POINT ( 'NONE',  ( -6.500000000000000000, 0.000000000000000000, 3.930000000000000160 ) ) ;
#32135=EDGE_CURVE ( 'NONE', #27961, #20453, #4730, .T. ) ;
#32166=CARTESIAN_POINT ( 'NONE',  ( 1.649999999999999911, 2.020667218593132262E-16, 0.000000000000000000 ) ) ;
#32228=CYLINDRICAL_SURFACE ( 'NONE', #1878, 1.999999999999999556 ) ;
#32294=PRODUCT_DEFINITION ( 'UNKNOWN', '', #15587, #24216 ) ;
#32349=FACE_OUTER_BOUND ( 'NONE', #30219, .T. ) ;
#32389=DIRECTION ( 'NONE',  ( 0.000000000000000000, 0.000000000000000000, 1.000000000000000000 ) ) ;
#32495=CARTESIAN_POINT ( 'NONE',  ( 0.000000000000000000, 0.000000000000000000, 3.180000000000000160 ) ) ;
#32736=ORIENTED_EDGE ( 'NONE', *, *, #26484, .T. ) ;
#32764=CARTESIAN_POINT ( 'NONE',  ( -4.875000000000000000, 2.702098422956710877, 0.000000000000000000 ) ) ;
#32791=LINE ( 'NONE', #8415, #12619 ) ;
#32815=CARTESIAN_POINT ( 'NONE',  ( -1.649999999999999911, 0.000000000000000000, 3.180000000000000160 ) ) ;
#32988=CARTESIAN_POINT ( 'NONE',  ( -6.500000000000000000, 0.000000000000000000, 0.000000000000000000 ) ) ;
#33055=VERTEX_POINT ( 'NONE', #24588 ) ;
#33082=EDGE_LOOP ( 'NONE', ( #3431, #16640, #26491, #24912 ) ) ;
#33103=VECTOR ( 'NONE', #30080, 1000.000000000000000 ) ;
#33126=ORIENTED_EDGE ( 'NONE', *, *, #682, .F. ) ;
#33175=DIRECTION ( 'NONE',  ( 0.000000000000000000, 0.000000000000000000, -1.000000000000000000 ) ) ;
#33180=CARTESIAN_POINT ( 'NONE',  ( -3.250000000000000000, -5.838643359331793015, 3.930000000000000160 ) ) ;
#33201=CARTESIAN_POINT ( 'NONE',  ( -5.344999999999999751, 1.414467053015192657E-16, -0.7500000000000000000 ) ) ;
#33239=CARTESIAN_POINT ( 'NONE',  ( -3.250000000000000000, 5.404196845913421754, -0.7500000000000000000 ) ) ;
#33286=VERTEX_POINT ( 'NONE', #17670 ) ;
#33347=DIRECTION ( 'NONE',  ( -1.000000000000000000, 0.000000000000000000, 0.000000000000000000 ) ) ;
#33369=CYLINDRICAL_SURFACE ( 'NONE', #28547, 1.154999999999999805 ) ;
#33393=DIRECTION ( 'NONE',  ( -0.000000000000000000, -0.000000000000000000, -1.000000000000000000 ) ) ;
#33401=VERTEX_POINT ( 'NONE', #10520 ) ;
#33426=ORIENTED_EDGE ( 'NONE', *, *, #9035, .T. ) ;
#33446=DIRECTION ( 'NONE',  ( 0.000000000000000000, 0.000000000000000000, -1.000000000000000000 ) ) ;
#33468=DIRECTION ( 'NONE',  ( -0.000000000000000000, -0.000000000000000000, 1.000000000000000000 ) ) ;
#33493=AXIS2_PLACEMENT_3D ( 'NONE', #24930, #30466, #6059 ) ;
#33596=CARTESIAN_POINT ( 'NONE',  ( 1.649999999999999911, 2.020667218593132262E-16, 3.180000000000000160 ) ) ;
#33660=VERTEX_POINT ( 'NONE', #17940 ) ;
#33675=ORIENTED_EDGE ( 'NONE', *, *, #2472, .F. ) ;
#33681=ORIENTED_EDGE ( 'NONE', *, *, #11972, .F. ) ;
#33699=ORIENTED_EDGE ( 'NONE', *, *, #30868, .T. ) ;
#33708=DIRECTION ( 'NONE',  ( 0.000000000000000000, 0.000000000000000000, 1.000000000000000000 ) ) ;
#33716=CARTESIAN_POINT ( 'NONE',  ( 0.000000000000000000, 0.000000000000000000, 3.930000000000000160 ) ) ;
#33770=DIRECTION ( 'NONE',  ( 1.000000000000000000, 0.000000000000000000, 0.000000000000000000 ) ) ;
#33803=CIRCLE ( 'NONE', #20719, 1.649999999999999911 ) ;
#33846=DIRECTION ( 'NONE',  ( 1.000000000000000000, 0.000000000000000000, 0.000000000000000000 ) ) ;
#33854=CARTESIAN_POINT ( 'NONE',  ( -0.6763010051031078662, -1.505030548027689319, 3.180000000000000160 ) ) ;
#33968=APPLICATION_CONTEXT ( 'automotive_design' ) ;
#33995=ORIENTED_EDGE ( 'NONE', *, *, #23625, .F. ) ;
#34070=AXIS2_PLACEMENT_3D ( 'NONE', #30517, #6282, #25158 ) ;
#34075=CIRCLE ( 'NONE', #1108, 4.306175033202026547 ) ;
#34102=EDGE_LOOP ( 'NONE', ( #8807, #14275, #23534, #27788 ) ) ;
#34116=DIRECTION ( 'NONE',  ( 1.000000000000000000, 0.000000000000000000, 0.000000000000000000 ) ) ;
#34195=DIRECTION ( 'NONE',  ( -0.000000000000000000, -0.000000000000000000, 1.000000000000000000 ) ) ;
#34207=ORIENTED_EDGE ( 'NONE', *, *, #16575, .F. ) ;
#34244=CARTESIAN_POINT ( 'NONE',  ( 0.000000000000000000, 0.000000000000000000, 3.180000000000000160 ) ) ;
#34248=ORIENTED_EDGE ( 'NONE', *, *, #8485, .F. ) ;
#34274=EDGE_CURVE ( 'NONE', #25337, #1716, #32791, .T. ) ;
#34284=DIRECTION ( 'NONE',  ( 0.000000000000000000, 0.000000000000000000, 1.000000000000000000 ) ) ;
#34329=AXIS2_PLACEMENT_3D ( 'NONE', #29161, #20632, #4756 ) ;
#34331=DIRECTION ( 'NONE',  ( -0.000000000000000000, -0.000000000000000000, 1.000000000000000000 ) ) ;
#34425=FACE_OUTER_BOUND ( 'NONE', #31438, .T. ) ;
#34454=ORIENTED_EDGE ( 'NONE', *, *, #34274, .F. ) ;
#34461=MECHANICAL_DESIGN_GEOMETRIC_PRESENTATION_REPRESENTATION('',(#23097),#17446);
#34467=ADVANCED_FACE ( 'NONE', ( #18372 ), #32228, .T. ) ;
#34483=ORIENTED_EDGE ( 'NONE', *, *, #9447, .F. ) ;
#34513=EDGE_LOOP ( 'NONE', ( #23727, #24117, #30094, #1435 ) ) ;
#34517=AXIS2_PLACEMENT_3D ( 'NONE', #28333, #4274, #33846 ) ;
#34539=CARTESIAN_POINT ( 'NONE',  ( -6.500000000000000000, 0.000000000000000000, 3.930000000000000160 ) ) ;
#34569=CARTESIAN_POINT ( 'NONE',  ( -0.9727285265192152641, -1.747512292859696670, -0.7500000000000000000 ) ) ;
#34593=AXIS2_PLACEMENT_3D ( 'NONE', #32764, #8557, #8389 ) ;
#34643=ORIENTED_EDGE ( 'NONE', *, *, #8995, .F. ) ;
#34714=AXIS2_PLACEMENT_3D ( 'NONE', #20499, #276, #18370 ) ;
#34774=CIRCLE ( 'NONE', #13181, 1.999999999999999112 ) ;
#34811=ORIENTED_EDGE ( 'NONE', *, *, #3324, .T. ) ;
#34955=CARTESIAN_POINT ( 'NONE',  ( -1.625000000000000000, 2.702098422956710877, 3.180000000000000160 ) ) ;
#34975=ORIENTED_EDGE ( 'NONE', *, *, #20454, .F. ) ;
#34981=VECTOR ( 'NONE', #9150, 1000.000000000000000 ) ;
#35049=EDGE_CURVE ( 'NONE', #7313, #12505, #11523, .T. ) ;
#35061=EDGE_CURVE ( 'NONE', #29588, #16280, #19905, .T. ) ;
#35074=ORIENTED_EDGE ( 'NONE', *, *, #40, .T. ) ;
#35075=VERTEX_POINT ( 'NONE', #22917 ) ;
#35283=COLOUR_RGB('Off White',0.89,0.88,0.83);
#35284=FILL_AREA_STYLE_COLOUR('',#35283);
#35285=FILL_AREA_STYLE('',(#35284));
#35286=SURFACE_STYLE_FILL_AREA(#35285);
#35287=SURFACE_SIDE_STYLE('',(#35286));
#35288=SURFACE_STYLE_USAGE(.BOTH.,#35287);
#35289=PRESENTATION_STYLE_ASSIGNMENT((#35288));
ENDSEC;
END-ISO-10303-21;
